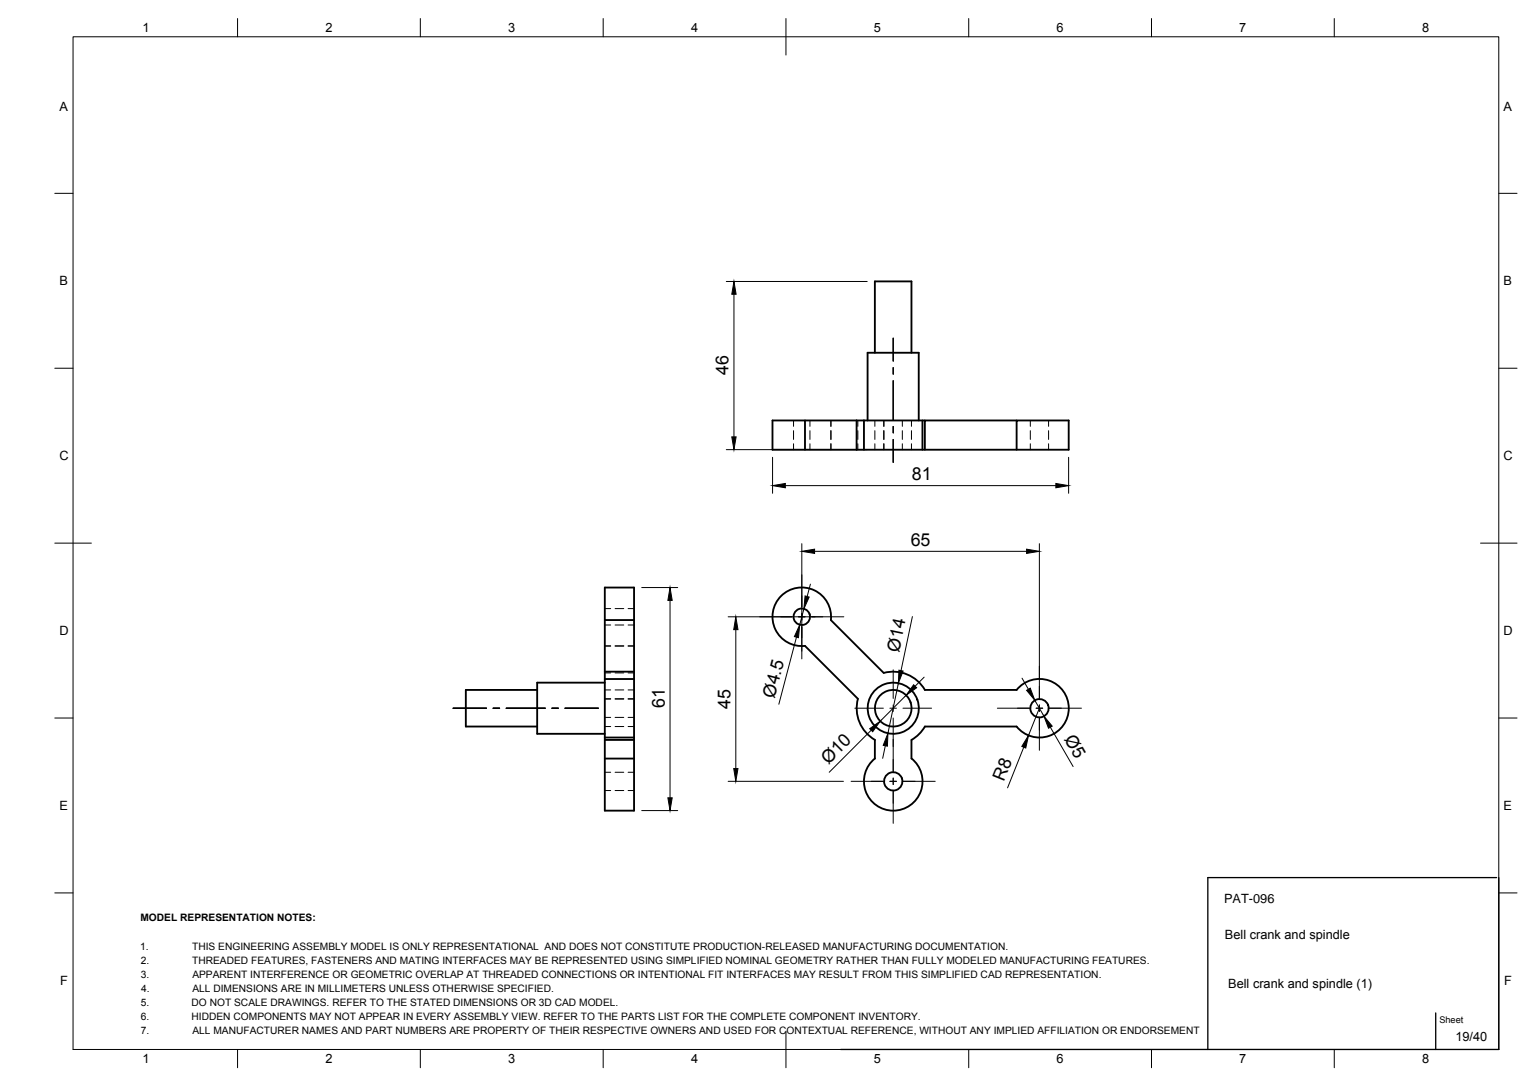
ISO-10303-21;
HEADER;
/* Generated by software containing ST-Developer
 * from STEP Tools, Inc. (www.steptools.com) 
 */

FILE_DESCRIPTION(
/* description */ ('PAT-096'),
/* implementation_level */ '2;1');

FILE_NAME(
/* name */ 'Bell crank and spindle.step',
/* time_stamp */ '2026-10-29T17:03:14-07:00',
/* author */ (''),
/* organization */ (''),
/* preprocessor_version */ 'ST-DEVELOPER v20.2',
/* originating_system */ 'Autodesk Translation Framework v15.17.0.0',
/* authorisation */ '');

FILE_SCHEMA (('AUTOMOTIVE_DESIGN { 1 0 10303 214 3 1 1 }'));
ENDSEC;

DATA;
#10=MECHANICAL_DESIGN_GEOMETRIC_PRESENTATION_REPRESENTATION('',(#418),#10650);
#348=SHAPE_REPRESENTATION_RELATIONSHIP('SRR','None',#10810,#379);
#379=ADVANCED_BREP_SHAPE_REPRESENTATION('',(#456),#10628);
#418=STYLED_ITEM('',(#11057),#456);
#456=MANIFOLD_SOLID_BREP('Body1',#5552);
#542=FACE_BOUND('',#1361,.T.);
#543=FACE_BOUND('',#1362,.T.);
#544=FACE_BOUND('',#1363,.T.);
#545=FACE_BOUND('',#1370,.T.);
#546=FACE_BOUND('',#1371,.T.);
#547=FACE_BOUND('',#1372,.T.);
#548=FACE_BOUND('',#1373,.T.);
#549=FACE_BOUND('',#1380,.T.);
#686=PLANE('',#6286);
#687=PLANE('',#6287);
#688=PLANE('',#6293);
#689=PLANE('',#6300);
#690=PLANE('',#6301);
#691=PLANE('',#6305);
#692=PLANE('',#6307);
#693=PLANE('',#6308);
#694=PLANE('',#6310);
#695=PLANE('',#6316);
#950=FACE_OUTER_BOUND('',#1355,.T.);
#951=FACE_OUTER_BOUND('',#1356,.T.);
#952=FACE_OUTER_BOUND('',#1357,.T.);
#953=FACE_OUTER_BOUND('',#1358,.T.);
#954=FACE_OUTER_BOUND('',#1359,.T.);
#955=FACE_OUTER_BOUND('',#1360,.T.);
#956=FACE_OUTER_BOUND('',#1364,.T.);
#957=FACE_OUTER_BOUND('',#1365,.T.);
#958=FACE_OUTER_BOUND('',#1366,.T.);
#959=FACE_OUTER_BOUND('',#1367,.T.);
#960=FACE_OUTER_BOUND('',#1368,.T.);
#961=FACE_OUTER_BOUND('',#1369,.T.);
#962=FACE_OUTER_BOUND('',#1374,.T.);
#963=FACE_OUTER_BOUND('',#1375,.T.);
#964=FACE_OUTER_BOUND('',#1376,.T.);
#965=FACE_OUTER_BOUND('',#1377,.T.);
#966=FACE_OUTER_BOUND('',#1378,.T.);
#967=FACE_OUTER_BOUND('',#1379,.T.);
#968=FACE_OUTER_BOUND('',#1381,.T.);
#969=FACE_OUTER_BOUND('',#1382,.T.);
#970=FACE_OUTER_BOUND('',#1383,.T.);
#1355=EDGE_LOOP('',(#4391,#4392,#4393,#4394));
#1356=EDGE_LOOP('',(#4395,#4396,#4397,#4398));
#1357=EDGE_LOOP('',(#4399,#4400,#4401,#4402));
#1358=EDGE_LOOP('',(#4403,#4404,#4405,#4406));
#1359=EDGE_LOOP('',(#4407,#4408,#4409,#4410));
#1360=EDGE_LOOP('',(#4411,#4412,#4413,#4414,#4415,#4416,#4417,#4418,#4419,
#4420,#4421,#4422));
#1361=EDGE_LOOP('',(#4423));
#1362=EDGE_LOOP('',(#4424));
#1363=EDGE_LOOP('',(#4425));
#1364=EDGE_LOOP('',(#4426,#4427,#4428,#4429));
#1365=EDGE_LOOP('',(#4430,#4431,#4432,#4433));
#1366=EDGE_LOOP('',(#4434,#4435,#4436,#4437));
#1367=EDGE_LOOP('',(#4438,#4439,#4440,#4441));
#1368=EDGE_LOOP('',(#4442,#4443,#4444,#4445));
#1369=EDGE_LOOP('',(#4446,#4447,#4448,#4449,#4450,#4451,#4452,#4453,#4454,
#4455,#4456,#4457));
#1370=EDGE_LOOP('',(#4458));
#1371=EDGE_LOOP('',(#4459));
#1372=EDGE_LOOP('',(#4460));
#1373=EDGE_LOOP('',(#4461));
#1374=EDGE_LOOP('',(#4462,#4463,#4464,#4465));
#1375=EDGE_LOOP('',(#4466,#4467,#4468,#4469));
#1376=EDGE_LOOP('',(#4470,#4471,#4472,#4473));
#1377=EDGE_LOOP('',(#4474,#4475,#4476,#4477));
#1378=EDGE_LOOP('',(#4478,#4479,#4480,#4481));
#1379=EDGE_LOOP('',(#4482));
#1380=EDGE_LOOP('',(#4483));
#1381=EDGE_LOOP('',(#4484,#4485,#4486,#4487));
#1382=EDGE_LOOP('',(#4488,#4489,#4490,#4491));
#1383=EDGE_LOOP('',(#4492));
#1736=LINE('',#9695,#2065);
#1737=LINE('',#9701,#2066);
#1738=LINE('',#9707,#2067);
#1739=LINE('',#9712,#2068);
#1740=LINE('',#9716,#2069);
#1741=LINE('',#9720,#2070);
#1742=LINE('',#9722,#2071);
#1743=LINE('',#9723,#2072);
#1744=LINE('',#9726,#2073);
#1745=LINE('',#9730,#2074);
#1746=LINE('',#9734,#2075);
#1747=LINE('',#9738,#2076);
#1748=LINE('',#9742,#2077);
#1749=LINE('',#9746,#2078);
#1750=LINE('',#9747,#2079);
#1751=LINE('',#9750,#2080);
#1752=LINE('',#9755,#2081);
#1753=LINE('',#9758,#2082);
#1754=LINE('',#9760,#2083);
#1755=LINE('',#9764,#2084);
#1756=LINE('',#9765,#2085);
#1757=LINE('',#9768,#2086);
#1758=LINE('',#9772,#2087);
#1759=LINE('',#9774,#2088);
#1760=LINE('',#9779,#2089);
#1761=LINE('',#9780,#2090);
#1762=LINE('',#9782,#2091);
#1763=LINE('',#9791,#2092);
#1764=LINE('',#9794,#2093);
#2065=VECTOR('',#7528,0.25);
#2066=VECTOR('',#7535,0.25);
#2067=VECTOR('',#7542,0.225);
#2068=VECTOR('',#7547,1.);
#2069=VECTOR('',#7550,1.);
#2070=VECTOR('',#7555,1.);
#2071=VECTOR('',#7556,1.);
#2072=VECTOR('',#7557,1.);
#2073=VECTOR('',#7560,1.);
#2074=VECTOR('',#7563,1.);
#2075=VECTOR('',#7566,1.);
#2076=VECTOR('',#7569,1.);
#2077=VECTOR('',#7572,1.);
#2078=VECTOR('',#7577,1.);
#2079=VECTOR('',#7578,1.);
#2080=VECTOR('',#7581,1.);
#2081=VECTOR('',#7588,1.);
#2082=VECTOR('',#7591,1.);
#2083=VECTOR('',#7592,1.);
#2084=VECTOR('',#7597,1.);
#2085=VECTOR('',#7598,1.);
#2086=VECTOR('',#7601,1.);
#2087=VECTOR('',#7604,1.);
#2088=VECTOR('',#7607,1.);
#2089=VECTOR('',#7614,1.);
#2090=VECTOR('',#7615,1.);
#2091=VECTOR('',#7618,1.);
#2092=VECTOR('',#7631,0.7);
#2093=VECTOR('',#7634,0.5);
#2436=CIRCLE('',#6275,0.25);
#2437=CIRCLE('',#6276,0.25);
#2438=CIRCLE('',#6278,0.25);
#2439=CIRCLE('',#6279,0.25);
#2440=CIRCLE('',#6281,0.225);
#2441=CIRCLE('',#6282,0.225);
#2442=CIRCLE('',#6284,0.8);
#2443=CIRCLE('',#6285,0.8);
#2444=CIRCLE('',#6288,1.);
#2445=CIRCLE('',#6289,0.8);
#2446=CIRCLE('',#6290,1.);
#2447=CIRCLE('',#6291,0.8);
#2448=CIRCLE('',#6292,1.);
#2449=CIRCLE('',#6295,1.);
#2450=CIRCLE('',#6297,1.);
#2451=CIRCLE('',#6299,0.8);
#2452=CIRCLE('',#6302,0.8);
#2453=CIRCLE('',#6303,1.);
#2454=CIRCLE('',#6304,0.7);
#2455=CIRCLE('',#6311,0.7);
#2456=CIRCLE('',#6312,0.5);
#2457=CIRCLE('',#6315,0.5);
#2811=VERTEX_POINT('',#9692);
#2812=VERTEX_POINT('',#9694);
#2813=VERTEX_POINT('',#9698);
#2814=VERTEX_POINT('',#9700);
#2815=VERTEX_POINT('',#9704);
#2816=VERTEX_POINT('',#9706);
#2817=VERTEX_POINT('',#9710);
#2818=VERTEX_POINT('',#9711);
#2819=VERTEX_POINT('',#9713);
#2820=VERTEX_POINT('',#9715);
#2821=VERTEX_POINT('',#9719);
#2822=VERTEX_POINT('',#9721);
#2823=VERTEX_POINT('',#9725);
#2824=VERTEX_POINT('',#9727);
#2825=VERTEX_POINT('',#9729);
#2826=VERTEX_POINT('',#9731);
#2827=VERTEX_POINT('',#9733);
#2828=VERTEX_POINT('',#9735);
#2829=VERTEX_POINT('',#9737);
#2830=VERTEX_POINT('',#9739);
#2831=VERTEX_POINT('',#9741);
#2832=VERTEX_POINT('',#9745);
#2833=VERTEX_POINT('',#9749);
#2834=VERTEX_POINT('',#9753);
#2835=VERTEX_POINT('',#9757);
#2836=VERTEX_POINT('',#9759);
#2837=VERTEX_POINT('',#9763);
#2838=VERTEX_POINT('',#9767);
#2839=VERTEX_POINT('',#9769);
#2840=VERTEX_POINT('',#9771);
#2841=VERTEX_POINT('',#9775);
#2842=VERTEX_POINT('',#9786);
#2843=VERTEX_POINT('',#9788);
#2844=VERTEX_POINT('',#9793);
#3374=EDGE_CURVE('',#2811,#2811,#2436,.T.);
#3375=EDGE_CURVE('',#2811,#2812,#1736,.T.);
#3376=EDGE_CURVE('',#2812,#2812,#2437,.T.);
#3377=EDGE_CURVE('',#2813,#2813,#2438,.T.);
#3378=EDGE_CURVE('',#2813,#2814,#1737,.T.);
#3379=EDGE_CURVE('',#2814,#2814,#2439,.T.);
#3380=EDGE_CURVE('',#2815,#2815,#2440,.T.);
#3381=EDGE_CURVE('',#2815,#2816,#1738,.T.);
#3382=EDGE_CURVE('',#2816,#2816,#2441,.T.);
#3383=EDGE_CURVE('',#2817,#2818,#1739,.T.);
#3384=EDGE_CURVE('',#2817,#2819,#2442,.T.);
#3385=EDGE_CURVE('',#2820,#2819,#1740,.T.);
#3386=EDGE_CURVE('',#2818,#2820,#2443,.T.);
#3387=EDGE_CURVE('',#2821,#2818,#1741,.T.);
#3388=EDGE_CURVE('',#2822,#2821,#1742,.T.);
#3389=EDGE_CURVE('',#2817,#2822,#1743,.T.);
#3390=EDGE_CURVE('',#2820,#2823,#1744,.T.);
#3391=EDGE_CURVE('',#2823,#2824,#2444,.T.);
#3392=EDGE_CURVE('',#2824,#2825,#1745,.T.);
#3393=EDGE_CURVE('',#2825,#2826,#2445,.T.);
#3394=EDGE_CURVE('',#2826,#2827,#1746,.T.);
#3395=EDGE_CURVE('',#2827,#2828,#2446,.T.);
#3396=EDGE_CURVE('',#2828,#2829,#1747,.T.);
#3397=EDGE_CURVE('',#2829,#2830,#2447,.T.);
#3398=EDGE_CURVE('',#2830,#2831,#1748,.T.);
#3399=EDGE_CURVE('',#2831,#2821,#2448,.T.);
#3400=EDGE_CURVE('',#2832,#2819,#1749,.T.);
#3401=EDGE_CURVE('',#2823,#2832,#1750,.T.);
#3402=EDGE_CURVE('',#2831,#2833,#1751,.T.);
#3403=EDGE_CURVE('',#2833,#2822,#2449,.T.);
#3404=EDGE_CURVE('',#2832,#2834,#2450,.T.);
#3405=EDGE_CURVE('',#2834,#2824,#1752,.T.);
#3406=EDGE_CURVE('',#2826,#2835,#1753,.T.);
#3407=EDGE_CURVE('',#2836,#2825,#1754,.T.);
#3408=EDGE_CURVE('',#2836,#2835,#2451,.T.);
#3409=EDGE_CURVE('',#2837,#2835,#1755,.T.);
#3410=EDGE_CURVE('',#2827,#2837,#1756,.T.);
#3411=EDGE_CURVE('',#2833,#2838,#1757,.T.);
#3412=EDGE_CURVE('',#2839,#2838,#2452,.T.);
#3413=EDGE_CURVE('',#2839,#2840,#1758,.T.);
#3414=EDGE_CURVE('',#2837,#2840,#2453,.T.);
#3415=EDGE_CURVE('',#2836,#2834,#1759,.T.);
#3416=EDGE_CURVE('',#2841,#2841,#2454,.T.);
#3417=EDGE_CURVE('',#2839,#2829,#1760,.T.);
#3418=EDGE_CURVE('',#2830,#2838,#1761,.T.);
#3419=EDGE_CURVE('',#2840,#2828,#1762,.T.);
#3420=EDGE_CURVE('',#2842,#2842,#2455,.T.);
#3421=EDGE_CURVE('',#2843,#2843,#2456,.T.);
#3422=EDGE_CURVE('',#2841,#2842,#1763,.T.);
#3423=EDGE_CURVE('',#2843,#2844,#1764,.T.);
#3424=EDGE_CURVE('',#2844,#2844,#2457,.T.);
#4391=ORIENTED_EDGE('',*,*,#3374,.F.);
#4392=ORIENTED_EDGE('',*,*,#3375,.T.);
#4393=ORIENTED_EDGE('',*,*,#3376,.F.);
#4394=ORIENTED_EDGE('',*,*,#3375,.F.);
#4395=ORIENTED_EDGE('',*,*,#3377,.F.);
#4396=ORIENTED_EDGE('',*,*,#3378,.T.);
#4397=ORIENTED_EDGE('',*,*,#3379,.F.);
#4398=ORIENTED_EDGE('',*,*,#3378,.F.);
#4399=ORIENTED_EDGE('',*,*,#3380,.F.);
#4400=ORIENTED_EDGE('',*,*,#3381,.T.);
#4401=ORIENTED_EDGE('',*,*,#3382,.F.);
#4402=ORIENTED_EDGE('',*,*,#3381,.F.);
#4403=ORIENTED_EDGE('',*,*,#3383,.F.);
#4404=ORIENTED_EDGE('',*,*,#3384,.T.);
#4405=ORIENTED_EDGE('',*,*,#3385,.F.);
#4406=ORIENTED_EDGE('',*,*,#3386,.F.);
#4407=ORIENTED_EDGE('',*,*,#3383,.T.);
#4408=ORIENTED_EDGE('',*,*,#3387,.F.);
#4409=ORIENTED_EDGE('',*,*,#3388,.F.);
#4410=ORIENTED_EDGE('',*,*,#3389,.F.);
#4411=ORIENTED_EDGE('',*,*,#3386,.T.);
#4412=ORIENTED_EDGE('',*,*,#3390,.T.);
#4413=ORIENTED_EDGE('',*,*,#3391,.T.);
#4414=ORIENTED_EDGE('',*,*,#3392,.T.);
#4415=ORIENTED_EDGE('',*,*,#3393,.T.);
#4416=ORIENTED_EDGE('',*,*,#3394,.T.);
#4417=ORIENTED_EDGE('',*,*,#3395,.T.);
#4418=ORIENTED_EDGE('',*,*,#3396,.T.);
#4419=ORIENTED_EDGE('',*,*,#3397,.T.);
#4420=ORIENTED_EDGE('',*,*,#3398,.T.);
#4421=ORIENTED_EDGE('',*,*,#3399,.T.);
#4422=ORIENTED_EDGE('',*,*,#3387,.T.);
#4423=ORIENTED_EDGE('',*,*,#3376,.T.);
#4424=ORIENTED_EDGE('',*,*,#3379,.T.);
#4425=ORIENTED_EDGE('',*,*,#3382,.T.);
#4426=ORIENTED_EDGE('',*,*,#3385,.T.);
#4427=ORIENTED_EDGE('',*,*,#3400,.F.);
#4428=ORIENTED_EDGE('',*,*,#3401,.F.);
#4429=ORIENTED_EDGE('',*,*,#3390,.F.);
#4430=ORIENTED_EDGE('',*,*,#3388,.T.);
#4431=ORIENTED_EDGE('',*,*,#3399,.F.);
#4432=ORIENTED_EDGE('',*,*,#3402,.T.);
#4433=ORIENTED_EDGE('',*,*,#3403,.T.);
#4434=ORIENTED_EDGE('',*,*,#3401,.T.);
#4435=ORIENTED_EDGE('',*,*,#3404,.T.);
#4436=ORIENTED_EDGE('',*,*,#3405,.T.);
#4437=ORIENTED_EDGE('',*,*,#3391,.F.);
#4438=ORIENTED_EDGE('',*,*,#3406,.F.);
#4439=ORIENTED_EDGE('',*,*,#3393,.F.);
#4440=ORIENTED_EDGE('',*,*,#3407,.F.);
#4441=ORIENTED_EDGE('',*,*,#3408,.T.);
#4442=ORIENTED_EDGE('',*,*,#3406,.T.);
#4443=ORIENTED_EDGE('',*,*,#3409,.F.);
#4444=ORIENTED_EDGE('',*,*,#3410,.F.);
#4445=ORIENTED_EDGE('',*,*,#3394,.F.);
#4446=ORIENTED_EDGE('',*,*,#3389,.T.);
#4447=ORIENTED_EDGE('',*,*,#3403,.F.);
#4448=ORIENTED_EDGE('',*,*,#3411,.T.);
#4449=ORIENTED_EDGE('',*,*,#3412,.F.);
#4450=ORIENTED_EDGE('',*,*,#3413,.T.);
#4451=ORIENTED_EDGE('',*,*,#3414,.F.);
#4452=ORIENTED_EDGE('',*,*,#3409,.T.);
#4453=ORIENTED_EDGE('',*,*,#3408,.F.);
#4454=ORIENTED_EDGE('',*,*,#3415,.T.);
#4455=ORIENTED_EDGE('',*,*,#3404,.F.);
#4456=ORIENTED_EDGE('',*,*,#3400,.T.);
#4457=ORIENTED_EDGE('',*,*,#3384,.F.);
#4458=ORIENTED_EDGE('',*,*,#3374,.T.);
#4459=ORIENTED_EDGE('',*,*,#3377,.T.);
#4460=ORIENTED_EDGE('',*,*,#3380,.T.);
#4461=ORIENTED_EDGE('',*,*,#3416,.T.);
#4462=ORIENTED_EDGE('',*,*,#3407,.T.);
#4463=ORIENTED_EDGE('',*,*,#3392,.F.);
#4464=ORIENTED_EDGE('',*,*,#3405,.F.);
#4465=ORIENTED_EDGE('',*,*,#3415,.F.);
#4466=ORIENTED_EDGE('',*,*,#3417,.F.);
#4467=ORIENTED_EDGE('',*,*,#3412,.T.);
#4468=ORIENTED_EDGE('',*,*,#3418,.F.);
#4469=ORIENTED_EDGE('',*,*,#3397,.F.);
#4470=ORIENTED_EDGE('',*,*,#3417,.T.);
#4471=ORIENTED_EDGE('',*,*,#3396,.F.);
#4472=ORIENTED_EDGE('',*,*,#3419,.F.);
#4473=ORIENTED_EDGE('',*,*,#3413,.F.);
#4474=ORIENTED_EDGE('',*,*,#3418,.T.);
#4475=ORIENTED_EDGE('',*,*,#3411,.F.);
#4476=ORIENTED_EDGE('',*,*,#3402,.F.);
#4477=ORIENTED_EDGE('',*,*,#3398,.F.);
#4478=ORIENTED_EDGE('',*,*,#3410,.T.);
#4479=ORIENTED_EDGE('',*,*,#3414,.T.);
#4480=ORIENTED_EDGE('',*,*,#3419,.T.);
#4481=ORIENTED_EDGE('',*,*,#3395,.F.);
#4482=ORIENTED_EDGE('',*,*,#3420,.F.);
#4483=ORIENTED_EDGE('',*,*,#3421,.F.);
#4484=ORIENTED_EDGE('',*,*,#3416,.F.);
#4485=ORIENTED_EDGE('',*,*,#3422,.T.);
#4486=ORIENTED_EDGE('',*,*,#3420,.T.);
#4487=ORIENTED_EDGE('',*,*,#3422,.F.);
#4488=ORIENTED_EDGE('',*,*,#3421,.T.);
#4489=ORIENTED_EDGE('',*,*,#3423,.T.);
#4490=ORIENTED_EDGE('',*,*,#3424,.T.);
#4491=ORIENTED_EDGE('',*,*,#3423,.F.);
#4492=ORIENTED_EDGE('',*,*,#3424,.F.);
#5131=CYLINDRICAL_SURFACE('',#6274,0.25);
#5132=CYLINDRICAL_SURFACE('',#6277,0.25);
#5133=CYLINDRICAL_SURFACE('',#6280,0.225);
#5134=CYLINDRICAL_SURFACE('',#6283,0.8);
#5135=CYLINDRICAL_SURFACE('',#6294,1.);
#5136=CYLINDRICAL_SURFACE('',#6296,1.);
#5137=CYLINDRICAL_SURFACE('',#6298,0.8);
#5138=CYLINDRICAL_SURFACE('',#6306,0.8);
#5139=CYLINDRICAL_SURFACE('',#6309,1.);
#5140=CYLINDRICAL_SURFACE('',#6313,0.7);
#5141=CYLINDRICAL_SURFACE('',#6314,0.5);
#5355=ADVANCED_FACE('',(#950),#5131,.F.);
#5356=ADVANCED_FACE('',(#951),#5132,.F.);
#5357=ADVANCED_FACE('',(#952),#5133,.F.);
#5358=ADVANCED_FACE('',(#953),#5134,.T.);
#5359=ADVANCED_FACE('',(#954),#686,.T.);
#5360=ADVANCED_FACE('',(#955,#542,#543,#544),#687,.T.);
#5361=ADVANCED_FACE('',(#956),#688,.T.);
#5362=ADVANCED_FACE('',(#957),#5135,.T.);
#5363=ADVANCED_FACE('',(#958),#5136,.T.);
#5364=ADVANCED_FACE('',(#959),#5137,.T.);
#5365=ADVANCED_FACE('',(#960),#689,.T.);
#5366=ADVANCED_FACE('',(#961,#545,#546,#547,#548),#690,.F.);
#5367=ADVANCED_FACE('',(#962),#691,.T.);
#5368=ADVANCED_FACE('',(#963),#5138,.T.);
#5369=ADVANCED_FACE('',(#964),#692,.T.);
#5370=ADVANCED_FACE('',(#965),#693,.T.);
#5371=ADVANCED_FACE('',(#966),#5139,.T.);
#5372=ADVANCED_FACE('',(#967,#549),#694,.F.);
#5373=ADVANCED_FACE('',(#968),#5140,.T.);
#5374=ADVANCED_FACE('',(#969),#5141,.T.);
#5375=ADVANCED_FACE('',(#970),#695,.F.);
#5552=CLOSED_SHELL('',(#5355,#5356,#5357,#5358,#5359,#5360,#5361,#5362,
#5363,#5364,#5365,#5366,#5367,#5368,#5369,#5370,#5371,#5372,#5373,#5374,
#5375));
#6273=AXIS2_PLACEMENT_3D('',#9690,#7522,#7523);
#6274=AXIS2_PLACEMENT_3D('',#9691,#7524,#7525);
#6275=AXIS2_PLACEMENT_3D('',#9693,#7526,#7527);
#6276=AXIS2_PLACEMENT_3D('',#9696,#7529,#7530);
#6277=AXIS2_PLACEMENT_3D('',#9697,#7531,#7532);
#6278=AXIS2_PLACEMENT_3D('',#9699,#7533,#7534);
#6279=AXIS2_PLACEMENT_3D('',#9702,#7536,#7537);
#6280=AXIS2_PLACEMENT_3D('',#9703,#7538,#7539);
#6281=AXIS2_PLACEMENT_3D('',#9705,#7540,#7541);
#6282=AXIS2_PLACEMENT_3D('',#9708,#7543,#7544);
#6283=AXIS2_PLACEMENT_3D('',#9709,#7545,#7546);
#6284=AXIS2_PLACEMENT_3D('',#9714,#7548,#7549);
#6285=AXIS2_PLACEMENT_3D('',#9717,#7551,#7552);
#6286=AXIS2_PLACEMENT_3D('',#9718,#7553,#7554);
#6287=AXIS2_PLACEMENT_3D('',#9724,#7558,#7559);
#6288=AXIS2_PLACEMENT_3D('',#9728,#7561,#7562);
#6289=AXIS2_PLACEMENT_3D('',#9732,#7564,#7565);
#6290=AXIS2_PLACEMENT_3D('',#9736,#7567,#7568);
#6291=AXIS2_PLACEMENT_3D('',#9740,#7570,#7571);
#6292=AXIS2_PLACEMENT_3D('',#9743,#7573,#7574);
#6293=AXIS2_PLACEMENT_3D('',#9744,#7575,#7576);
#6294=AXIS2_PLACEMENT_3D('',#9748,#7579,#7580);
#6295=AXIS2_PLACEMENT_3D('',#9751,#7582,#7583);
#6296=AXIS2_PLACEMENT_3D('',#9752,#7584,#7585);
#6297=AXIS2_PLACEMENT_3D('',#9754,#7586,#7587);
#6298=AXIS2_PLACEMENT_3D('',#9756,#7589,#7590);
#6299=AXIS2_PLACEMENT_3D('',#9761,#7593,#7594);
#6300=AXIS2_PLACEMENT_3D('',#9762,#7595,#7596);
#6301=AXIS2_PLACEMENT_3D('',#9766,#7599,#7600);
#6302=AXIS2_PLACEMENT_3D('',#9770,#7602,#7603);
#6303=AXIS2_PLACEMENT_3D('',#9773,#7605,#7606);
#6304=AXIS2_PLACEMENT_3D('',#9776,#7608,#7609);
#6305=AXIS2_PLACEMENT_3D('',#9777,#7610,#7611);
#6306=AXIS2_PLACEMENT_3D('',#9778,#7612,#7613);
#6307=AXIS2_PLACEMENT_3D('',#9781,#7616,#7617);
#6308=AXIS2_PLACEMENT_3D('',#9783,#7619,#7620);
#6309=AXIS2_PLACEMENT_3D('',#9784,#7621,#7622);
#6310=AXIS2_PLACEMENT_3D('',#9785,#7623,#7624);
#6311=AXIS2_PLACEMENT_3D('',#9787,#7625,#7626);
#6312=AXIS2_PLACEMENT_3D('',#9789,#7627,#7628);
#6313=AXIS2_PLACEMENT_3D('',#9790,#7629,#7630);
#6314=AXIS2_PLACEMENT_3D('',#9792,#7632,#7633);
#6315=AXIS2_PLACEMENT_3D('',#9795,#7635,#7636);
#6316=AXIS2_PLACEMENT_3D('',#9796,#7637,#7638);
#7522=DIRECTION('axis',(0.,0.,1.));
#7523=DIRECTION('refdir',(1.,0.,0.));
#7524=DIRECTION('center_axis',(0.,0.,1.));
#7525=DIRECTION('ref_axis',(1.,0.,0.));
#7526=DIRECTION('center_axis',(0.,0.,1.));
#7527=DIRECTION('ref_axis',(1.,0.,0.));
#7528=DIRECTION('',(0.,0.,1.));
#7529=DIRECTION('center_axis',(0.,0.,-1.));
#7530=DIRECTION('ref_axis',(1.,0.,0.));
#7531=DIRECTION('center_axis',(0.,0.,1.));
#7532=DIRECTION('ref_axis',(1.,0.,0.));
#7533=DIRECTION('center_axis',(0.,0.,1.));
#7534=DIRECTION('ref_axis',(1.,0.,0.));
#7535=DIRECTION('',(0.,0.,1.));
#7536=DIRECTION('center_axis',(0.,0.,-1.));
#7537=DIRECTION('ref_axis',(1.,0.,0.));
#7538=DIRECTION('center_axis',(0.,0.,1.));
#7539=DIRECTION('ref_axis',(1.,0.,0.));
#7540=DIRECTION('center_axis',(0.,0.,1.));
#7541=DIRECTION('ref_axis',(1.,0.,0.));
#7542=DIRECTION('',(0.,0.,1.));
#7543=DIRECTION('center_axis',(0.,0.,-1.));
#7544=DIRECTION('ref_axis',(1.,0.,0.));
#7545=DIRECTION('center_axis',(0.,0.,1.));
#7546=DIRECTION('ref_axis',(-0.707106781186548,-0.707106781186547,0.));
#7547=DIRECTION('',(0.,0.,1.));
#7548=DIRECTION('center_axis',(0.,0.,1.));
#7549=DIRECTION('ref_axis',(1.,0.,0.));
#7550=DIRECTION('',(0.,0.,-1.));
#7551=DIRECTION('center_axis',(0.,0.,1.));
#7552=DIRECTION('ref_axis',(1.,0.,0.));
#7553=DIRECTION('center_axis',(-0.707106781186548,0.707106781186548,0.));
#7554=DIRECTION('ref_axis',(-0.707106781186548,-0.707106781186548,0.));
#7555=DIRECTION('',(-0.707106781186548,-0.707106781186548,0.));
#7556=DIRECTION('',(0.,0.,1.));
#7557=DIRECTION('',(0.707106781186548,0.707106781186548,0.));
#7558=DIRECTION('center_axis',(0.,0.,1.));
#7559=DIRECTION('ref_axis',(1.,0.,0.));
#7560=DIRECTION('',(0.707106781186548,0.707106781186548,0.));
#7561=DIRECTION('center_axis',(0.,0.,1.));
#7562=DIRECTION('ref_axis',(1.,0.,0.));
#7563=DIRECTION('',(1.,0.,0.));
#7564=DIRECTION('center_axis',(0.,0.,1.));
#7565=DIRECTION('ref_axis',(1.,0.,0.));
#7566=DIRECTION('',(-1.,0.,0.));
#7567=DIRECTION('center_axis',(0.,0.,1.));
#7568=DIRECTION('ref_axis',(1.,0.,0.));
#7569=DIRECTION('',(0.,1.,0.));
#7570=DIRECTION('center_axis',(0.,0.,1.));
#7571=DIRECTION('ref_axis',(1.,0.,0.));
#7572=DIRECTION('',(0.,-1.,0.));
#7573=DIRECTION('center_axis',(0.,0.,1.));
#7574=DIRECTION('ref_axis',(1.,0.,0.));
#7575=DIRECTION('center_axis',(0.707106781186548,-0.707106781186548,0.));
#7576=DIRECTION('ref_axis',(0.707106781186548,0.707106781186548,0.));
#7577=DIRECTION('',(-0.707106781186548,-0.707106781186548,0.));
#7578=DIRECTION('',(0.,0.,-1.));
#7579=DIRECTION('center_axis',(0.,0.,1.));
#7580=DIRECTION('ref_axis',(-0.923879532511287,0.38268343236509,0.));
#7581=DIRECTION('',(0.,0.,-1.));
#7582=DIRECTION('center_axis',(0.,0.,1.));
#7583=DIRECTION('ref_axis',(1.,0.,0.));
#7584=DIRECTION('center_axis',(0.,0.,1.));
#7585=DIRECTION('ref_axis',(1.,0.,0.));
#7586=DIRECTION('center_axis',(0.,0.,1.));
#7587=DIRECTION('ref_axis',(1.,0.,0.));
#7588=DIRECTION('',(0.,0.,1.));
#7589=DIRECTION('center_axis',(0.,0.,1.));
#7590=DIRECTION('ref_axis',(1.,0.,0.));
#7591=DIRECTION('',(0.,0.,-1.));
#7592=DIRECTION('',(0.,0.,1.));
#7593=DIRECTION('center_axis',(0.,0.,1.));
#7594=DIRECTION('ref_axis',(1.,0.,0.));
#7595=DIRECTION('center_axis',(0.,1.,0.));
#7596=DIRECTION('ref_axis',(-1.,0.,0.));
#7597=DIRECTION('',(1.,0.,0.));
#7598=DIRECTION('',(0.,0.,-1.));
#7599=DIRECTION('center_axis',(0.,0.,1.));
#7600=DIRECTION('ref_axis',(1.,0.,0.));
#7601=DIRECTION('',(0.,1.,0.));
#7602=DIRECTION('center_axis',(0.,0.,1.));
#7603=DIRECTION('ref_axis',(1.,0.,0.));
#7604=DIRECTION('',(0.,-1.,0.));
#7605=DIRECTION('center_axis',(0.,0.,1.));
#7606=DIRECTION('ref_axis',(1.,0.,0.));
#7607=DIRECTION('',(-1.,0.,0.));
#7608=DIRECTION('center_axis',(0.,0.,1.));
#7609=DIRECTION('ref_axis',(1.,0.,0.));
#7610=DIRECTION('center_axis',(0.,-1.,0.));
#7611=DIRECTION('ref_axis',(1.,0.,0.));
#7612=DIRECTION('center_axis',(0.,0.,1.));
#7613=DIRECTION('ref_axis',(6.12323399573677E-17,1.,0.));
#7614=DIRECTION('',(0.,0.,1.));
#7615=DIRECTION('',(0.,0.,-1.));
#7616=DIRECTION('center_axis',(1.,0.,0.));
#7617=DIRECTION('ref_axis',(0.,1.,0.));
#7618=DIRECTION('',(0.,0.,1.));
#7619=DIRECTION('center_axis',(-1.,0.,0.));
#7620=DIRECTION('ref_axis',(0.,-1.,0.));
#7621=DIRECTION('center_axis',(0.,0.,1.));
#7622=DIRECTION('ref_axis',(1.,0.,0.));
#7623=DIRECTION('center_axis',(0.,0.,1.));
#7624=DIRECTION('ref_axis',(1.,0.,0.));
#7625=DIRECTION('center_axis',(0.,0.,1.));
#7626=DIRECTION('ref_axis',(1.,0.,0.));
#7627=DIRECTION('center_axis',(0.,0.,-1.));
#7628=DIRECTION('ref_axis',(1.,0.,0.));
#7629=DIRECTION('center_axis',(0.,0.,1.));
#7630=DIRECTION('ref_axis',(1.,0.,0.));
#7631=DIRECTION('',(0.,0.,-1.));
#7632=DIRECTION('center_axis',(0.,0.,1.));
#7633=DIRECTION('ref_axis',(1.,0.,0.));
#7634=DIRECTION('',(0.,0.,-1.));
#7635=DIRECTION('center_axis',(0.,0.,1.));
#7636=DIRECTION('ref_axis',(1.,0.,0.));
#7637=DIRECTION('center_axis',(0.,0.,1.));
#7638=DIRECTION('ref_axis',(1.,0.,0.));
#9690=CARTESIAN_POINT('',(0.,0.,0.));
#9691=CARTESIAN_POINT('Origin',(4.,0.,4.7));
#9692=CARTESIAN_POINT('',(3.75,-3.06161699786838E-17,4.8));
#9693=CARTESIAN_POINT('Origin',(4.,0.,4.8));
#9694=CARTESIAN_POINT('',(3.75,3.06161699786838E-17,5.6));
#9695=CARTESIAN_POINT('',(3.75,-3.06161699786838E-17,4.7));
#9696=CARTESIAN_POINT('Origin',(4.,0.,5.6));
#9697=CARTESIAN_POINT('Origin',(0.,2.,4.7));
#9698=CARTESIAN_POINT('',(-0.25,2.,4.8));
#9699=CARTESIAN_POINT('Origin',(0.,2.,4.8));
#9700=CARTESIAN_POINT('',(-0.25,2.,5.6));
#9701=CARTESIAN_POINT('',(-0.25,2.,4.7));
#9702=CARTESIAN_POINT('Origin',(0.,2.,5.6));
#9703=CARTESIAN_POINT('Origin',(-2.5,-2.5,4.7));
#9704=CARTESIAN_POINT('',(-2.725,-2.5,4.8));
#9705=CARTESIAN_POINT('Origin',(-2.5,-2.5,4.8));
#9706=CARTESIAN_POINT('',(-2.725,-2.5,5.6));
#9707=CARTESIAN_POINT('',(-2.725,-2.5,4.7));
#9708=CARTESIAN_POINT('Origin',(-2.5,-2.5,5.6));
#9709=CARTESIAN_POINT('Origin',(-2.5,-2.5,4.8));
#9710=CARTESIAN_POINT('',(-2.41196534727688,-1.70485856609033,4.8));
#9711=CARTESIAN_POINT('',(-2.41196534727688,-1.70485856609033,5.6));
#9712=CARTESIAN_POINT('',(-2.41196534727688,-1.70485856609033,4.8));
#9713=CARTESIAN_POINT('',(-1.70485856609033,-2.41196534727688,4.8));
#9714=CARTESIAN_POINT('Origin',(-2.5,-2.5,4.8));
#9715=CARTESIAN_POINT('',(-1.70485856609033,-2.41196534727688,5.6));
#9716=CARTESIAN_POINT('',(-1.70485856609033,-2.41196534727688,4.8));
#9717=CARTESIAN_POINT('Origin',(-2.5,-2.5,5.6));
#9718=CARTESIAN_POINT('Origin',(-0.353553390593274,0.353553390593274,4.8));
#9719=CARTESIAN_POINT('',(-0.965925826289068,-0.25881904510252,5.6));
#9720=CARTESIAN_POINT('',(-2.85355339059327,-2.14644660940673,5.6));
#9721=CARTESIAN_POINT('',(-0.965925826289068,-0.258819045102521,4.8));
#9722=CARTESIAN_POINT('',(-0.965925826289068,-0.258819045102521,4.8));
#9723=CARTESIAN_POINT('',(-2.85355339059327,-2.14644660940673,4.8));
#9724=CARTESIAN_POINT('Origin',(0.,0.,5.6));
#9725=CARTESIAN_POINT('',(-0.258819045102521,-0.965925826289068,5.6));
#9726=CARTESIAN_POINT('',(0.353553390593274,-0.353553390593274,5.6));
#9727=CARTESIAN_POINT('',(0.866025403784439,-0.5,5.6));
#9728=CARTESIAN_POINT('Origin',(0.,0.,5.6));
#9729=CARTESIAN_POINT('',(3.37550020016016,-0.5,5.6));
#9730=CARTESIAN_POINT('',(4.,-0.5,5.6));
#9731=CARTESIAN_POINT('',(3.37550020016016,0.5,5.6));
#9732=CARTESIAN_POINT('Origin',(4.,0.,5.6));
#9733=CARTESIAN_POINT('',(0.866025403784439,0.5,5.6));
#9734=CARTESIAN_POINT('',(0.,0.5,5.6));
#9735=CARTESIAN_POINT('',(0.5,0.866025403784439,5.6));
#9736=CARTESIAN_POINT('Origin',(0.,0.,5.6));
#9737=CARTESIAN_POINT('',(0.5,1.37550020016016,5.6));
#9738=CARTESIAN_POINT('',(0.5,2.,5.6));
#9739=CARTESIAN_POINT('',(-0.5,1.37550020016016,5.6));
#9740=CARTESIAN_POINT('Origin',(0.,2.,5.6));
#9741=CARTESIAN_POINT('',(-0.5,0.866025403784439,5.6));
#9742=CARTESIAN_POINT('',(-0.5,0.,5.6));
#9743=CARTESIAN_POINT('Origin',(0.,0.,5.6));
#9744=CARTESIAN_POINT('Origin',(-2.14644660940673,-2.85355339059327,4.8));
#9745=CARTESIAN_POINT('',(-0.25881904510252,-0.965925826289068,4.8));
#9746=CARTESIAN_POINT('',(0.353553390593274,-0.353553390593274,4.8));
#9747=CARTESIAN_POINT('',(-0.25881904510252,-0.965925826289068,4.8));
#9748=CARTESIAN_POINT('Origin',(0.,0.,4.8));
#9749=CARTESIAN_POINT('',(-0.5,0.866025403784439,4.8));
#9750=CARTESIAN_POINT('',(-0.5,0.866025403784439,4.8));
#9751=CARTESIAN_POINT('Origin',(0.,0.,4.8));
#9752=CARTESIAN_POINT('Origin',(0.,0.,4.8));
#9753=CARTESIAN_POINT('',(0.866025403784439,-0.5,4.8));
#9754=CARTESIAN_POINT('Origin',(0.,0.,4.8));
#9755=CARTESIAN_POINT('',(0.866025403784439,-0.5,4.8));
#9756=CARTESIAN_POINT('Origin',(4.,0.,4.8));
#9757=CARTESIAN_POINT('',(3.37550020016016,0.5,4.8));
#9758=CARTESIAN_POINT('',(3.37550020016016,0.5,4.8));
#9759=CARTESIAN_POINT('',(3.37550020016016,-0.5,4.8));
#9760=CARTESIAN_POINT('',(3.37550020016016,-0.5,4.8));
#9761=CARTESIAN_POINT('Origin',(4.,0.,4.8));
#9762=CARTESIAN_POINT('Origin',(4.,0.5,4.8));
#9763=CARTESIAN_POINT('',(0.866025403784439,0.5,4.8));
#9764=CARTESIAN_POINT('',(0.,0.5,4.8));
#9765=CARTESIAN_POINT('',(0.866025403784439,0.5,4.8));
#9766=CARTESIAN_POINT('Origin',(0.,0.,4.8));
#9767=CARTESIAN_POINT('',(-0.5,1.37550020016016,4.8));
#9768=CARTESIAN_POINT('',(-0.5,0.,4.8));
#9769=CARTESIAN_POINT('',(0.5,1.37550020016016,4.8));
#9770=CARTESIAN_POINT('Origin',(0.,2.,4.8));
#9771=CARTESIAN_POINT('',(0.5,0.866025403784439,4.8));
#9772=CARTESIAN_POINT('',(0.5,2.,4.8));
#9773=CARTESIAN_POINT('Origin',(0.,0.,4.8));
#9774=CARTESIAN_POINT('',(4.,-0.5,4.8));
#9775=CARTESIAN_POINT('',(-0.7,-8.57252759403147E-17,4.8));
#9776=CARTESIAN_POINT('Origin',(0.,0.,4.8));
#9777=CARTESIAN_POINT('Origin',(0.,-0.5,4.8));
#9778=CARTESIAN_POINT('Origin',(0.,2.,4.8));
#9779=CARTESIAN_POINT('',(0.5,1.37550020016016,4.8));
#9780=CARTESIAN_POINT('',(-0.5,1.37550020016016,4.8));
#9781=CARTESIAN_POINT('Origin',(0.5,0.,4.8));
#9782=CARTESIAN_POINT('',(0.5,0.866025403784439,4.8));
#9783=CARTESIAN_POINT('Origin',(-0.5,2.,4.8));
#9784=CARTESIAN_POINT('Origin',(0.,0.,4.8));
#9785=CARTESIAN_POINT('Origin',(0.,0.,2.95));
#9786=CARTESIAN_POINT('',(-0.7,-8.57252759403147E-17,2.95));
#9787=CARTESIAN_POINT('Origin',(0.,0.,2.95));
#9788=CARTESIAN_POINT('',(-0.5,6.12323399573677E-17,2.95));
#9789=CARTESIAN_POINT('Origin',(0.,0.,2.95));
#9790=CARTESIAN_POINT('Origin',(0.,0.,2.95));
#9791=CARTESIAN_POINT('',(-0.7,-8.57252759403147E-17,2.95));
#9792=CARTESIAN_POINT('Origin',(0.,0.,1.));
#9793=CARTESIAN_POINT('',(-0.5,-6.12323399573677E-17,1.));
#9794=CARTESIAN_POINT('',(-0.5,-6.12323399573677E-17,1.));
#9795=CARTESIAN_POINT('Origin',(0.,0.,1.));
#9796=CARTESIAN_POINT('Origin',(0.,0.,1.));
#10589=UNCERTAINTY_MEASURE_WITH_UNIT(LENGTH_MEASURE(0.001),#10651,
'DISTANCE_ACCURACY_VALUE',
'Maximum model space distance between geometric entities at asserted c
onnectivities');
#10611=UNCERTAINTY_MEASURE_WITH_UNIT(LENGTH_MEASURE(0.001),#10651,
'DISTANCE_ACCURACY_VALUE',
'Maximum model space distance between geometric entities at asserted c
onnectivities');
#10628=(
GEOMETRIC_REPRESENTATION_CONTEXT(3)
GLOBAL_UNCERTAINTY_ASSIGNED_CONTEXT((#10589))
GLOBAL_UNIT_ASSIGNED_CONTEXT((#10651,#10653,#10654))
REPRESENTATION_CONTEXT('','3D')
);
#10650=(
GEOMETRIC_REPRESENTATION_CONTEXT(3)
GLOBAL_UNCERTAINTY_ASSIGNED_CONTEXT((#10611))
GLOBAL_UNIT_ASSIGNED_CONTEXT((#10651,#10653,#10654))
REPRESENTATION_CONTEXT('','3D')
);
#10651=(
LENGTH_UNIT()
NAMED_UNIT(*)
SI_UNIT(.CENTI.,.METRE.)
);
#10653=(
NAMED_UNIT(*)
PLANE_ANGLE_UNIT()
SI_UNIT($,.RADIAN.)
);
#10654=(
NAMED_UNIT(*)
SI_UNIT($,.STERADIAN.)
SOLID_ANGLE_UNIT()
);
#10671=SHAPE_DEFINITION_REPRESENTATION(#10714,#10810);
#10714=PRODUCT_DEFINITION_SHAPE('',$,#10849);
#10810=SHAPE_REPRESENTATION('',(#6273),#10628);
#10832=PRODUCT_DEFINITION_CONTEXT('part definition',#10948,'design');
#10849=PRODUCT_DEFINITION('Bell crank and spindle',
'Bell crank and spindle',#10887,#10832);
#10887=PRODUCT_DEFINITION_FORMATION('',$,#10966);
#10948=APPLICATION_CONTEXT(
'Core Data for Automotive Mechanical Design Process');
#10949=PRODUCT_CONTEXT('part definition',#10948,'mechanical');
#10966=PRODUCT('Bell crank and spindle','Bell crank and spindle',
'Bell crank and spindle',(#10949));
#11051=COLOUR_RGB('Sky Blue',0.24,0.69,0.87);
#11052=FILL_AREA_STYLE_COLOUR('',#11051);
#11053=FILL_AREA_STYLE('',(#11052));
#11054=SURFACE_STYLE_FILL_AREA(#11053);
#11055=SURFACE_SIDE_STYLE('',(#11054));
#11056=SURFACE_STYLE_USAGE(.BOTH.,#11055);
#11057=PRESENTATION_STYLE_ASSIGNMENT((#11056));
ENDSEC;
END-ISO-10303-21;
